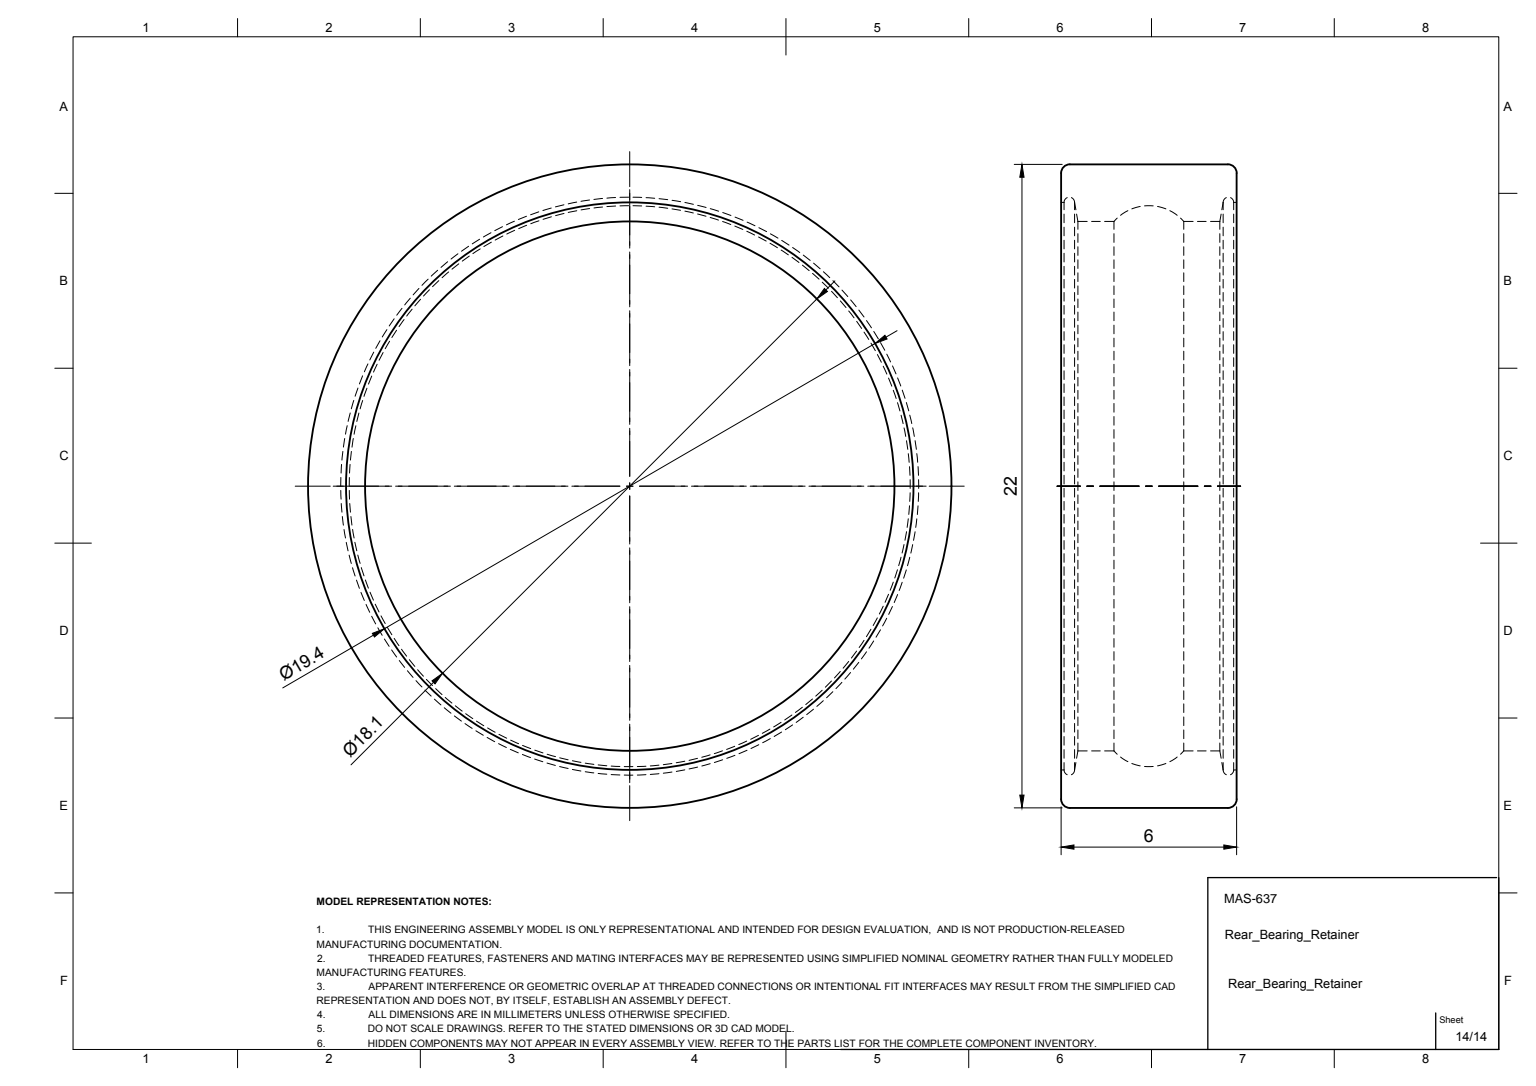
ISO-10303-21;
HEADER;
FILE_DESCRIPTION((''),'2;1');
FILE_NAME('Rear_Bearing_Retainer.step','2026-10-09T10:11:57-07:00',(''),(''),'','','');
FILE_SCHEMA (('AUTOMOTIVE_DESIGN { 1 0 10303 214 3 1 1 }'));
ENDSEC;
DATA;
#10=MECHANICAL_DESIGN_GEOMETRIC_PRESENTATION_REPRESENTATION('',(#154),#13510);
#107=SHAPE_REPRESENTATION_RELATIONSHIP('SRR','None',#13577,#122) ;
#122=ADVANCED_BREP_SHAPE_REPRESENTATION('',(#186),#13509) ;
#154=STYLED_ITEM('',(#13650),#186) ;
#186=MANIFOLD_SOLID_BREP('Body1',#7403) ;
#264=FACE_BOUND('',#1643,.T.) ;
#265=FACE_BOUND('',#1645,.T.) ;
#472=PLANE('',#8544) ;
#473=PLANE('',#8545) ;
#536=TOROIDAL_SURFACE('',#8522,9.7,0.18) ;
#537=TOROIDAL_SURFACE('',#8527,10.7,0.3) ;
#538=TOROIDAL_SURFACE('',#8533,10.7,0.3) ;
#539=TOROIDAL_SURFACE('',#8539,9.7,0.18) ;
#540=TOROIDAL_SURFACE('',#8550,8.,1.59) ;
#663=CYLINDRICAL_SURFACE('',#8525,9.7) ;
#664=CYLINDRICAL_SURFACE('',#8531,11.) ;
#665=CYLINDRICAL_SURFACE('',#8536,9.7) ;
#666=CYLINDRICAL_SURFACE('',#8546,9.05) ;
#667=CYLINDRICAL_SURFACE('',#8548,9.05) ;
#1108=FACE_OUTER_BOUND('',#1633,.T.) ;
#1109=FACE_OUTER_BOUND('',#1634,.T.) ;
#1110=FACE_OUTER_BOUND('',#1635,.T.) ;
#1111=FACE_OUTER_BOUND('',#1636,.T.) ;
#1112=FACE_OUTER_BOUND('',#1637,.T.) ;
#1113=FACE_OUTER_BOUND('',#1638,.T.) ;
#1114=FACE_OUTER_BOUND('',#1639,.T.) ;
#1115=FACE_OUTER_BOUND('',#1640,.T.) ;
#1116=FACE_OUTER_BOUND('',#1641,.T.) ;
#1117=FACE_OUTER_BOUND('',#1642,.T.) ;
#1118=FACE_OUTER_BOUND('',#1644,.T.) ;
#1119=FACE_OUTER_BOUND('',#1646,.T.) ;
#1120=FACE_OUTER_BOUND('',#1647,.T.) ;
#1121=FACE_OUTER_BOUND('',#1648,.T.) ;
#1633=EDGE_LOOP('',(#6818,#6819,#6820,#6821)) ;
#1634=EDGE_LOOP('',(#6822,#6823,#6824,#6825)) ;
#1635=EDGE_LOOP('',(#6826,#6827,#6828,#6829)) ;
#1636=EDGE_LOOP('',(#6830,#6831,#6832,#6833)) ;
#1637=EDGE_LOOP('',(#6834,#6835,#6836,#6837)) ;
#1638=EDGE_LOOP('',(#6838,#6839,#6840,#6841)) ;
#1639=EDGE_LOOP('',(#6842,#6843,#6844,#6845)) ;
#1640=EDGE_LOOP('',(#6846,#6847,#6848,#6849)) ;
#1641=EDGE_LOOP('',(#6850,#6851,#6852,#6853)) ;
#1642=EDGE_LOOP('',(#6854)) ;
#1643=EDGE_LOOP('',(#6855)) ;
#1644=EDGE_LOOP('',(#6856)) ;
#1645=EDGE_LOOP('',(#6857)) ;
#1646=EDGE_LOOP('',(#6858,#6859,#6860,#6861)) ;
#1647=EDGE_LOOP('',(#6862,#6863,#6864,#6865)) ;
#1648=EDGE_LOOP('',(#6866,#6867,#6868,#6869)) ;
#2136=LINE('',#13412,#2630) ;
#2137=LINE('',#13421,#2631) ;
#2138=LINE('',#13431,#2632) ;
#2139=LINE('',#13440,#2633) ;
#2140=LINE('',#13449,#2634) ;
#2141=LINE('',#13455,#2635) ;
#2142=LINE('',#13458,#2636) ;
#2630=VECTOR('',#10956,9.05) ;
#2631=VECTOR('',#10969,9.7) ;
#2632=VECTOR('',#10982,11.) ;
#2633=VECTOR('',#10993,9.7) ;
#2634=VECTOR('',#11006,9.05) ;
#2635=VECTOR('',#11015,9.05) ;
#2636=VECTOR('',#11018,9.05) ;
#3124=CIRCLE('',#8520,9.05) ;
#3125=CIRCLE('',#8521,9.7) ;
#3126=CIRCLE('',#8523,9.7) ;
#3127=CIRCLE('',#8524,0.18) ;
#3128=CIRCLE('',#8526,9.7) ;
#3129=CIRCLE('',#8528,11.) ;
#3130=CIRCLE('',#8529,0.3) ;
#3131=CIRCLE('',#8530,10.7) ;
#3132=CIRCLE('',#8532,11.) ;
#3133=CIRCLE('',#8534,10.7) ;
#3134=CIRCLE('',#8535,0.3) ;
#3135=CIRCLE('',#8537,9.7) ;
#3136=CIRCLE('',#8538,9.7) ;
#3137=CIRCLE('',#8540,9.7) ;
#3138=CIRCLE('',#8541,0.18) ;
#3139=CIRCLE('',#8543,9.05) ;
#3140=CIRCLE('',#8547,9.05) ;
#3141=CIRCLE('',#8549,9.05) ;
#3142=CIRCLE('',#8551,1.59) ;
#3784=VERTEX_POINT('',#13409) ;
#3785=VERTEX_POINT('',#13411) ;
#3786=VERTEX_POINT('',#13415) ;
#3787=VERTEX_POINT('',#13419) ;
#3788=VERTEX_POINT('',#13423) ;
#3789=VERTEX_POINT('',#13425) ;
#3790=VERTEX_POINT('',#13429) ;
#3791=VERTEX_POINT('',#13433) ;
#3792=VERTEX_POINT('',#13437) ;
#3793=VERTEX_POINT('',#13439) ;
#3794=VERTEX_POINT('',#13443) ;
#3795=VERTEX_POINT('',#13447) ;
#3796=VERTEX_POINT('',#13453) ;
#3797=VERTEX_POINT('',#13457) ;
#4796=EDGE_CURVE('',#3784,#3784,#3124,.F.) ;
#4797=EDGE_CURVE('',#3784,#3785,#2136,.T.) ;
#4798=EDGE_CURVE('',#3785,#3785,#3125,.F.) ;
#4799=EDGE_CURVE('',#3786,#3786,#3126,.T.) ;
#4800=EDGE_CURVE('',#3786,#3785,#3127,.T.) ;
#4801=EDGE_CURVE('',#3787,#3787,#3128,.T.) ;
#4802=EDGE_CURVE('',#3787,#3786,#2137,.T.) ;
#4803=EDGE_CURVE('',#3788,#3788,#3129,.T.) ;
#4804=EDGE_CURVE('',#3788,#3789,#3130,.T.) ;
#4805=EDGE_CURVE('',#3789,#3789,#3131,.T.) ;
#4806=EDGE_CURVE('',#3790,#3790,#3132,.T.) ;
#4807=EDGE_CURVE('',#3790,#3788,#2138,.T.) ;
#4808=EDGE_CURVE('',#3791,#3791,#3133,.T.) ;
#4809=EDGE_CURVE('',#3791,#3790,#3134,.T.) ;
#4810=EDGE_CURVE('',#3792,#3792,#3135,.T.) ;
#4811=EDGE_CURVE('',#3792,#3793,#2139,.T.) ;
#4812=EDGE_CURVE('',#3793,#3793,#3136,.T.) ;
#4813=EDGE_CURVE('',#3794,#3794,#3137,.T.) ;
#4814=EDGE_CURVE('',#3794,#3792,#3138,.T.) ;
#4815=EDGE_CURVE('',#3795,#3795,#3139,.T.) ;
#4816=EDGE_CURVE('',#3795,#3794,#2140,.T.) ;
#4817=EDGE_CURVE('',#3796,#3796,#3140,.T.) ;
#4818=EDGE_CURVE('',#3796,#3795,#2141,.T.) ;
#4819=EDGE_CURVE('',#3784,#3797,#2142,.T.) ;
#4820=EDGE_CURVE('',#3797,#3797,#3141,.T.) ;
#4821=EDGE_CURVE('',#3797,#3796,#3142,.T.) ;
#6818=ORIENTED_EDGE('',*,*,#4796,.T.) ;
#6819=ORIENTED_EDGE('',*,*,#4797,.T.) ;
#6820=ORIENTED_EDGE('',*,*,#4798,.F.) ;
#6821=ORIENTED_EDGE('',*,*,#4797,.F.) ;
#6822=ORIENTED_EDGE('',*,*,#4799,.F.) ;
#6823=ORIENTED_EDGE('',*,*,#4800,.T.) ;
#6824=ORIENTED_EDGE('',*,*,#4798,.T.) ;
#6825=ORIENTED_EDGE('',*,*,#4800,.F.) ;
#6826=ORIENTED_EDGE('',*,*,#4801,.F.) ;
#6827=ORIENTED_EDGE('',*,*,#4802,.T.) ;
#6828=ORIENTED_EDGE('',*,*,#4799,.T.) ;
#6829=ORIENTED_EDGE('',*,*,#4802,.F.) ;
#6830=ORIENTED_EDGE('',*,*,#4803,.F.) ;
#6831=ORIENTED_EDGE('',*,*,#4804,.T.) ;
#6832=ORIENTED_EDGE('',*,*,#4805,.T.) ;
#6833=ORIENTED_EDGE('',*,*,#4804,.F.) ;
#6834=ORIENTED_EDGE('',*,*,#4806,.F.) ;
#6835=ORIENTED_EDGE('',*,*,#4807,.T.) ;
#6836=ORIENTED_EDGE('',*,*,#4803,.T.) ;
#6837=ORIENTED_EDGE('',*,*,#4807,.F.) ;
#6838=ORIENTED_EDGE('',*,*,#4808,.F.) ;
#6839=ORIENTED_EDGE('',*,*,#4809,.T.) ;
#6840=ORIENTED_EDGE('',*,*,#4806,.T.) ;
#6841=ORIENTED_EDGE('',*,*,#4809,.F.) ;
#6842=ORIENTED_EDGE('',*,*,#4810,.F.) ;
#6843=ORIENTED_EDGE('',*,*,#4811,.T.) ;
#6844=ORIENTED_EDGE('',*,*,#4812,.T.) ;
#6845=ORIENTED_EDGE('',*,*,#4811,.F.) ;
#6846=ORIENTED_EDGE('',*,*,#4813,.F.) ;
#6847=ORIENTED_EDGE('',*,*,#4814,.T.) ;
#6848=ORIENTED_EDGE('',*,*,#4810,.T.) ;
#6849=ORIENTED_EDGE('',*,*,#4814,.F.) ;
#6850=ORIENTED_EDGE('',*,*,#4815,.F.) ;
#6851=ORIENTED_EDGE('',*,*,#4816,.T.) ;
#6852=ORIENTED_EDGE('',*,*,#4813,.T.) ;
#6853=ORIENTED_EDGE('',*,*,#4816,.F.) ;
#6854=ORIENTED_EDGE('',*,*,#4805,.F.) ;
#6855=ORIENTED_EDGE('',*,*,#4801,.T.) ;
#6856=ORIENTED_EDGE('',*,*,#4808,.T.) ;
#6857=ORIENTED_EDGE('',*,*,#4812,.F.) ;
#6858=ORIENTED_EDGE('',*,*,#4817,.F.) ;
#6859=ORIENTED_EDGE('',*,*,#4818,.T.) ;
#6860=ORIENTED_EDGE('',*,*,#4815,.T.) ;
#6861=ORIENTED_EDGE('',*,*,#4818,.F.) ;
#6862=ORIENTED_EDGE('',*,*,#4796,.F.) ;
#6863=ORIENTED_EDGE('',*,*,#4819,.T.) ;
#6864=ORIENTED_EDGE('',*,*,#4820,.T.) ;
#6865=ORIENTED_EDGE('',*,*,#4819,.F.) ;
#6866=ORIENTED_EDGE('',*,*,#4820,.F.) ;
#6867=ORIENTED_EDGE('',*,*,#4821,.T.) ;
#6868=ORIENTED_EDGE('',*,*,#4817,.T.) ;
#6869=ORIENTED_EDGE('',*,*,#4821,.F.) ;
#6916=CONICAL_SURFACE('',#8519,9.05,1.3962634016) ;
#6917=CONICAL_SURFACE('',#8542,9.05,1.3962634016) ;
#7358=ADVANCED_FACE('',(#1108),#6916,.F.) ;
#7359=ADVANCED_FACE('',(#1109),#536,.F.) ;
#7360=ADVANCED_FACE('',(#1110),#663,.F.) ;
#7361=ADVANCED_FACE('',(#1111),#537,.T.) ;
#7362=ADVANCED_FACE('',(#1112),#664,.T.) ;
#7363=ADVANCED_FACE('',(#1113),#538,.T.) ;
#7364=ADVANCED_FACE('',(#1114),#665,.F.) ;
#7365=ADVANCED_FACE('',(#1115),#539,.F.) ;
#7366=ADVANCED_FACE('',(#1116),#6917,.F.) ;
#7367=ADVANCED_FACE('',(#1117,#264),#472,.F.) ;
#7368=ADVANCED_FACE('',(#1118,#265),#473,.T.) ;
#7369=ADVANCED_FACE('',(#1119),#666,.F.) ;
#7370=ADVANCED_FACE('',(#1120),#667,.F.) ;
#7371=ADVANCED_FACE('',(#1121),#540,.F.) ;
#7403=CLOSED_SHELL('',(#7358,#7359,#7360,#7361,#7362,#7363,#7364,#7365,
#7366,#7367,#7368,#7369,#7370,#7371)) ;
#8518=AXIS2_PLACEMENT_3D('',#13407,#10950,#10951) ;
#8519=AXIS2_PLACEMENT_3D('',#13408,#10952,#10953) ;
#8520=AXIS2_PLACEMENT_3D('',#13410,#10954,#10955) ;
#8521=AXIS2_PLACEMENT_3D('',#13413,#10957,#10958) ;
#8522=AXIS2_PLACEMENT_3D('',#13414,#10959,#10960) ;
#8523=AXIS2_PLACEMENT_3D('',#13416,#10961,#10962) ;
#8524=AXIS2_PLACEMENT_3D('',#13417,#10963,#10964) ;
#8525=AXIS2_PLACEMENT_3D('',#13418,#10965,#10966) ;
#8526=AXIS2_PLACEMENT_3D('',#13420,#10967,#10968) ;
#8527=AXIS2_PLACEMENT_3D('',#13422,#10970,#10971) ;
#8528=AXIS2_PLACEMENT_3D('',#13424,#10972,#10973) ;
#8529=AXIS2_PLACEMENT_3D('',#13426,#10974,#10975) ;
#8530=AXIS2_PLACEMENT_3D('',#13427,#10976,#10977) ;
#8531=AXIS2_PLACEMENT_3D('',#13428,#10978,#10979) ;
#8532=AXIS2_PLACEMENT_3D('',#13430,#10980,#10981) ;
#8533=AXIS2_PLACEMENT_3D('',#13432,#10983,#10984) ;
#8534=AXIS2_PLACEMENT_3D('',#13434,#10985,#10986) ;
#8535=AXIS2_PLACEMENT_3D('',#13435,#10987,#10988) ;
#8536=AXIS2_PLACEMENT_3D('',#13436,#10989,#10990) ;
#8537=AXIS2_PLACEMENT_3D('',#13438,#10991,#10992) ;
#8538=AXIS2_PLACEMENT_3D('',#13441,#10994,#10995) ;
#8539=AXIS2_PLACEMENT_3D('',#13442,#10996,#10997) ;
#8540=AXIS2_PLACEMENT_3D('',#13444,#10998,#10999) ;
#8541=AXIS2_PLACEMENT_3D('',#13445,#11000,#11001) ;
#8542=AXIS2_PLACEMENT_3D('',#13446,#11002,#11003) ;
#8543=AXIS2_PLACEMENT_3D('',#13448,#11004,#11005) ;
#8544=AXIS2_PLACEMENT_3D('',#13450,#11007,#11008) ;
#8545=AXIS2_PLACEMENT_3D('',#13451,#11009,#11010) ;
#8546=AXIS2_PLACEMENT_3D('',#13452,#11011,#11012) ;
#8547=AXIS2_PLACEMENT_3D('',#13454,#11013,#11014) ;
#8548=AXIS2_PLACEMENT_3D('',#13456,#11016,#11017) ;
#8549=AXIS2_PLACEMENT_3D('',#13459,#11019,#11020) ;
#8550=AXIS2_PLACEMENT_3D('',#13460,#11021,#11022) ;
#8551=AXIS2_PLACEMENT_3D('',#13461,#11023,#11024) ;
#10950=DIRECTION('axis',(0.,0.,1.)) ;
#10951=DIRECTION('refdir',(1.,0.,0.)) ;
#10952=DIRECTION('center_axis',(0.,0.,1.)) ;
#10953=DIRECTION('ref_axis',(0.877582561890372,-0.479425538604204,0.)) ;
#10954=DIRECTION('center_axis',(0.,0.,1.)) ;
#10955=DIRECTION('ref_axis',(-1.,0.,0.)) ;
#10956=DIRECTION('',(-0.864250110858646,0.472141987409851,0.173648177662463)) ;
#10957=DIRECTION('center_axis',(0.,0.,1.)) ;
#10958=DIRECTION('ref_axis',(-1.,0.,0.)) ;
#10959=DIRECTION('center_axis',(0.,0.,-1.)) ;
#10960=DIRECTION('ref_axis',(0.877582561890372,-0.479425538604204,0.)) ;
#10961=DIRECTION('center_axis',(0.,0.,-1.)) ;
#10962=DIRECTION('ref_axis',(1.,0.,0.)) ;
#10963=DIRECTION('center_axis',(-0.479425538604204,-0.877582561890372,0.)) ;
#10964=DIRECTION('ref_axis',(-0.877582561890372,0.479425538604204,0.)) ;
#10965=DIRECTION('center_axis',(0.,0.,-1.)) ;
#10966=DIRECTION('ref_axis',(0.877582561890372,-0.479425538604204,0.)) ;
#10967=DIRECTION('center_axis',(0.,0.,-1.)) ;
#10968=DIRECTION('ref_axis',(1.,0.,0.)) ;
#10969=DIRECTION('',(0.,0.,-1.)) ;
#10970=DIRECTION('center_axis',(0.,0.,-1.)) ;
#10971=DIRECTION('ref_axis',(0.877582561890372,-0.479425538604204,0.)) ;
#10972=DIRECTION('center_axis',(0.,0.,-1.)) ;
#10973=DIRECTION('ref_axis',(1.,0.,0.)) ;
#10974=DIRECTION('center_axis',(0.479425538604204,0.877582561890372,0.)) ;
#10975=DIRECTION('ref_axis',(-0.877582561890372,0.479425538604204,0.)) ;
#10976=DIRECTION('center_axis',(0.,0.,-1.)) ;
#10977=DIRECTION('ref_axis',(1.,0.,0.)) ;
#10978=DIRECTION('center_axis',(0.,0.,-1.)) ;
#10979=DIRECTION('ref_axis',(0.877582561890372,-0.479425538604204,0.)) ;
#10980=DIRECTION('center_axis',(0.,0.,-1.)) ;
#10981=DIRECTION('ref_axis',(1.,0.,0.)) ;
#10982=DIRECTION('',(0.,0.,1.)) ;
#10983=DIRECTION('center_axis',(0.,0.,-1.)) ;
#10984=DIRECTION('ref_axis',(0.877582561890372,-0.479425538604204,0.)) ;
#10985=DIRECTION('center_axis',(0.,0.,-1.)) ;
#10986=DIRECTION('ref_axis',(1.,0.,0.)) ;
#10987=DIRECTION('center_axis',(0.479425538604204,0.877582561890372,0.)) ;
#10988=DIRECTION('ref_axis',(-0.877582561890372,0.479425538604204,0.)) ;
#10989=DIRECTION('center_axis',(0.,0.,-1.)) ;
#10990=DIRECTION('ref_axis',(0.877582561890372,-0.479425538604204,0.)) ;
#10991=DIRECTION('center_axis',(0.,0.,-1.)) ;
#10992=DIRECTION('ref_axis',(1.,0.,0.)) ;
#10993=DIRECTION('',(0.,0.,-1.)) ;
#10994=DIRECTION('center_axis',(0.,0.,-1.)) ;
#10995=DIRECTION('ref_axis',(1.,0.,0.)) ;
#10996=DIRECTION('center_axis',(0.,0.,-1.)) ;
#10997=DIRECTION('ref_axis',(0.877582561890372,-0.479425538604204,0.)) ;
#10998=DIRECTION('center_axis',(0.,0.,-1.)) ;
#10999=DIRECTION('ref_axis',(1.,0.,0.)) ;
#11000=DIRECTION('center_axis',(-0.479425538604204,-0.877582561890372,0.)) ;
#11001=DIRECTION('ref_axis',(-0.877582561890372,0.479425538604204,0.)) ;
#11002=DIRECTION('center_axis',(0.,0.,-1.)) ;
#11003=DIRECTION('ref_axis',(0.877582561890372,-0.479425538604204,0.)) ;
#11004=DIRECTION('center_axis',(0.,0.,-1.)) ;
#11005=DIRECTION('ref_axis',(1.,0.,0.)) ;
#11006=DIRECTION('',(-0.864250110858646,0.472141987409852,-0.173648177662463)) ;
#11007=DIRECTION('center_axis',(0.,0.,-1.)) ;
#11008=DIRECTION('ref_axis',(1.,0.,0.)) ;
#11009=DIRECTION('center_axis',(0.,0.,-1.)) ;
#11010=DIRECTION('ref_axis',(1.,0.,0.)) ;
#11011=DIRECTION('center_axis',(0.,0.,-1.)) ;
#11012=DIRECTION('ref_axis',(0.877582561890372,-0.479425538604204,0.)) ;
#11013=DIRECTION('center_axis',(0.,0.,-1.)) ;
#11014=DIRECTION('ref_axis',(1.,0.,0.)) ;
#11015=DIRECTION('',(0.,0.,-1.)) ;
#11016=DIRECTION('center_axis',(0.,0.,-1.)) ;
#11017=DIRECTION('ref_axis',(0.877582561890372,-0.479425538604204,0.)) ;
#11018=DIRECTION('',(0.,0.,-1.)) ;
#11019=DIRECTION('center_axis',(0.,0.,-1.)) ;
#11020=DIRECTION('ref_axis',(1.,0.,0.)) ;
#11021=DIRECTION('center_axis',(0.,0.,-1.)) ;
#11022=DIRECTION('ref_axis',(0.877582561890372,-0.479425538604204,0.)) ;
#11023=DIRECTION('center_axis',(-0.479425538604204,-0.877582561890372,0.)) ;
#11024=DIRECTION('ref_axis',(-0.877582561890372,0.479425538604204,0.)) ;
#13407=CARTESIAN_POINT('',(0.,0.,0.)) ;
#13408=CARTESIAN_POINT('Origin',(0.,0.,114.425387463)) ;
#13409=CARTESIAN_POINT('',(-7.94212218510787,4.33880112436804,114.425387463)) ;
#13410=CARTESIAN_POINT('Origin',(0.,0.,114.425387463)) ;
#13411=CARTESIAN_POINT('',(-8.51255085026796,4.65042772442327,114.540000000444)) ;
#13412=CARTESIAN_POINT('',(-7.94212218510787,4.33880112436805,114.425387463)) ;
#13413=CARTESIAN_POINT('Origin',(0.,0.,114.54)) ;
#13414=CARTESIAN_POINT('Origin',(0.,0.,114.72)) ;
#13415=CARTESIAN_POINT('',(-8.51255085033661,4.65042772446077,114.9)) ;
#13416=CARTESIAN_POINT('Origin',(0.,0.,114.9)) ;
#13417=CARTESIAN_POINT('Origin',(-8.51255085033661,4.65042772446078,114.72)) ;
#13418=CARTESIAN_POINT('Origin',(0.,0.,112.)) ;
#13419=CARTESIAN_POINT('',(-8.51255085033661,4.65042772446077,115.)) ;
#13420=CARTESIAN_POINT('Origin',(0.,0.,115.)) ;
#13421=CARTESIAN_POINT('',(-8.51255085033661,4.65042772446078,112.)) ;
#13422=CARTESIAN_POINT('Origin',(0.,0.,114.7)) ;
#13423=CARTESIAN_POINT('',(-9.6534081807941,5.27368092464624,114.7)) ;
#13424=CARTESIAN_POINT('Origin',(0.,0.,114.7)) ;
#13425=CARTESIAN_POINT('',(-9.39013341222698,5.12985326306498,115.)) ;
#13426=CARTESIAN_POINT('Origin',(-9.39013341222698,5.12985326306499,114.7)) ;
#13427=CARTESIAN_POINT('Origin',(0.,0.,115.)) ;
#13428=CARTESIAN_POINT('Origin',(0.,0.,112.)) ;
#13429=CARTESIAN_POINT('',(-9.6534081807941,5.27368092464624,109.3)) ;
#13430=CARTESIAN_POINT('Origin',(0.,0.,109.3)) ;
#13431=CARTESIAN_POINT('',(-9.6534081807941,5.27368092464625,112.)) ;
#13432=CARTESIAN_POINT('Origin',(0.,0.,109.3)) ;
#13433=CARTESIAN_POINT('',(-9.39013341222698,5.12985326306498,109.)) ;
#13434=CARTESIAN_POINT('Origin',(0.,0.,109.)) ;
#13435=CARTESIAN_POINT('Origin',(-9.39013341222698,5.12985326306499,109.3)) ;
#13436=CARTESIAN_POINT('Origin',(0.,0.,112.)) ;
#13437=CARTESIAN_POINT('',(-8.51255085033661,4.65042772446077,109.1)) ;
#13438=CARTESIAN_POINT('Origin',(0.,0.,109.1)) ;
#13439=CARTESIAN_POINT('',(-8.51255085033661,4.65042772446077,109.)) ;
#13440=CARTESIAN_POINT('',(-8.51255085033661,4.65042772446078,112.)) ;
#13441=CARTESIAN_POINT('Origin',(0.,0.,109.)) ;
#13442=CARTESIAN_POINT('Origin',(0.,0.,109.28)) ;
#13443=CARTESIAN_POINT('',(-8.51255085033661,4.65042772446077,109.46)) ;
#13444=CARTESIAN_POINT('Origin',(0.,0.,109.46)) ;
#13445=CARTESIAN_POINT('Origin',(-8.51255085033661,4.65042772446078,109.28)) ;
#13446=CARTESIAN_POINT('Origin',(0.,0.,109.574612537)) ;
#13447=CARTESIAN_POINT('',(-7.94212218510787,4.33880112436804,109.574612537)) ;
#13448=CARTESIAN_POINT('Origin',(0.,0.,109.574612537)) ;
#13449=CARTESIAN_POINT('',(-7.94212218510787,4.33880112436805,109.574612537)) ;
#13450=CARTESIAN_POINT('Origin',(5.3,0.,115.)) ;
#13451=CARTESIAN_POINT('Origin',(5.3,0.,109.)) ;
#13452=CARTESIAN_POINT('Origin',(0.,0.,112.)) ;
#13453=CARTESIAN_POINT('',(-7.94212218511,4.33880112437,110.806015075)) ;
#13454=CARTESIAN_POINT('Origin',(0.,0.,110.806015075)) ;
#13455=CARTESIAN_POINT('',(-7.94212218510787,4.33880112436805,112.)) ;
#13456=CARTESIAN_POINT('Origin',(0.,0.,112.)) ;
#13457=CARTESIAN_POINT('',(-7.94212218511,4.33880112437,113.193984925)) ;
#13458=CARTESIAN_POINT('',(-7.94212218510787,4.33880112436805,112.)) ;
#13459=CARTESIAN_POINT('Origin',(0.,0.,113.193984925)) ;
#13460=CARTESIAN_POINT('Origin',(0.,0.,112.)) ;
#13461=CARTESIAN_POINT('Origin',(-7.02066049512298,3.83540430883363,112.)) ;
#13492=UNCERTAINTY_MEASURE_WITH_UNIT(LENGTH_MEASURE(0.01),#13511,
'DISTANCE_ACCURACY_VALUE',
'Maximum model space distance between geometric entities at asserted c
onnectivities') ;
#13493=UNCERTAINTY_MEASURE_WITH_UNIT(LENGTH_MEASURE(0.01),#13511,
'DISTANCE_ACCURACY_VALUE',
'Maximum model space distance between geometric entities at asserted c
onnectivities') ;
#13509=(
GEOMETRIC_REPRESENTATION_CONTEXT(3)
GLOBAL_UNCERTAINTY_ASSIGNED_CONTEXT((#13492))
GLOBAL_UNIT_ASSIGNED_CONTEXT((#13511,#13513,#13514))
REPRESENTATION_CONTEXT('','3D')
) ;
#13510=(
GEOMETRIC_REPRESENTATION_CONTEXT(3)
GLOBAL_UNCERTAINTY_ASSIGNED_CONTEXT((#13493))
GLOBAL_UNIT_ASSIGNED_CONTEXT((#13511,#13513,#13514))
REPRESENTATION_CONTEXT('','3D')
) ;
#13511=(
LENGTH_UNIT()
NAMED_UNIT(*)
SI_UNIT(.MILLI.,.METRE.)
) ;
#13513=(
NAMED_UNIT(*)
PLANE_ANGLE_UNIT()
SI_UNIT($,.RADIAN.)
) ;
#13514=(
NAMED_UNIT(*)
SI_UNIT($,.STERADIAN.)
SOLID_ANGLE_UNIT()
) ;
#13530=SHAPE_DEFINITION_REPRESENTATION(#13546,#13577) ;
#13546=PRODUCT_DEFINITION_SHAPE('',$,#13594) ;
#13577=SHAPE_REPRESENTATION('',(#8518),#13509) ;
#13578=PRODUCT_DEFINITION_CONTEXT('part definition',#13628,'design') ;
#13594=PRODUCT_DEFINITION('Rear_Bearing_Retainer',
'Rear_Bearing_Retainer',#13610,#13578) ;
#13610=PRODUCT_DEFINITION_FORMATION('',$,#13645) ;
#13628=APPLICATION_CONTEXT(
'Core Data for Automotive Mechanical Design Process') ;
#13629=PRODUCT_CONTEXT('part definition',#13628,'mechanical') ;
#13645=PRODUCT('Rear_Bearing_Retainer','Rear_Bearing_Retainer',$,(#13629)) ;
#13650=PRESENTATION_STYLE_ASSIGNMENT((#13655)) ;
#13655=SURFACE_STYLE_USAGE(.BOTH.,#13660) ;
#13660=SURFACE_SIDE_STYLE('',(#13665)) ;
#13665=SURFACE_STYLE_FILL_AREA(#13670) ;
#13670=FILL_AREA_STYLE('Opaque(144,144,144)',(#13675)) ;
#13675=FILL_AREA_STYLE_COLOUR('Opaque(144,144,144)',#13680) ;
#13680=COLOUR_RGB('Opaque(144,144,144)', 0.40784314, 0.44705882, 0.49803922) ;
ENDSEC;
END-ISO-10303-21;
